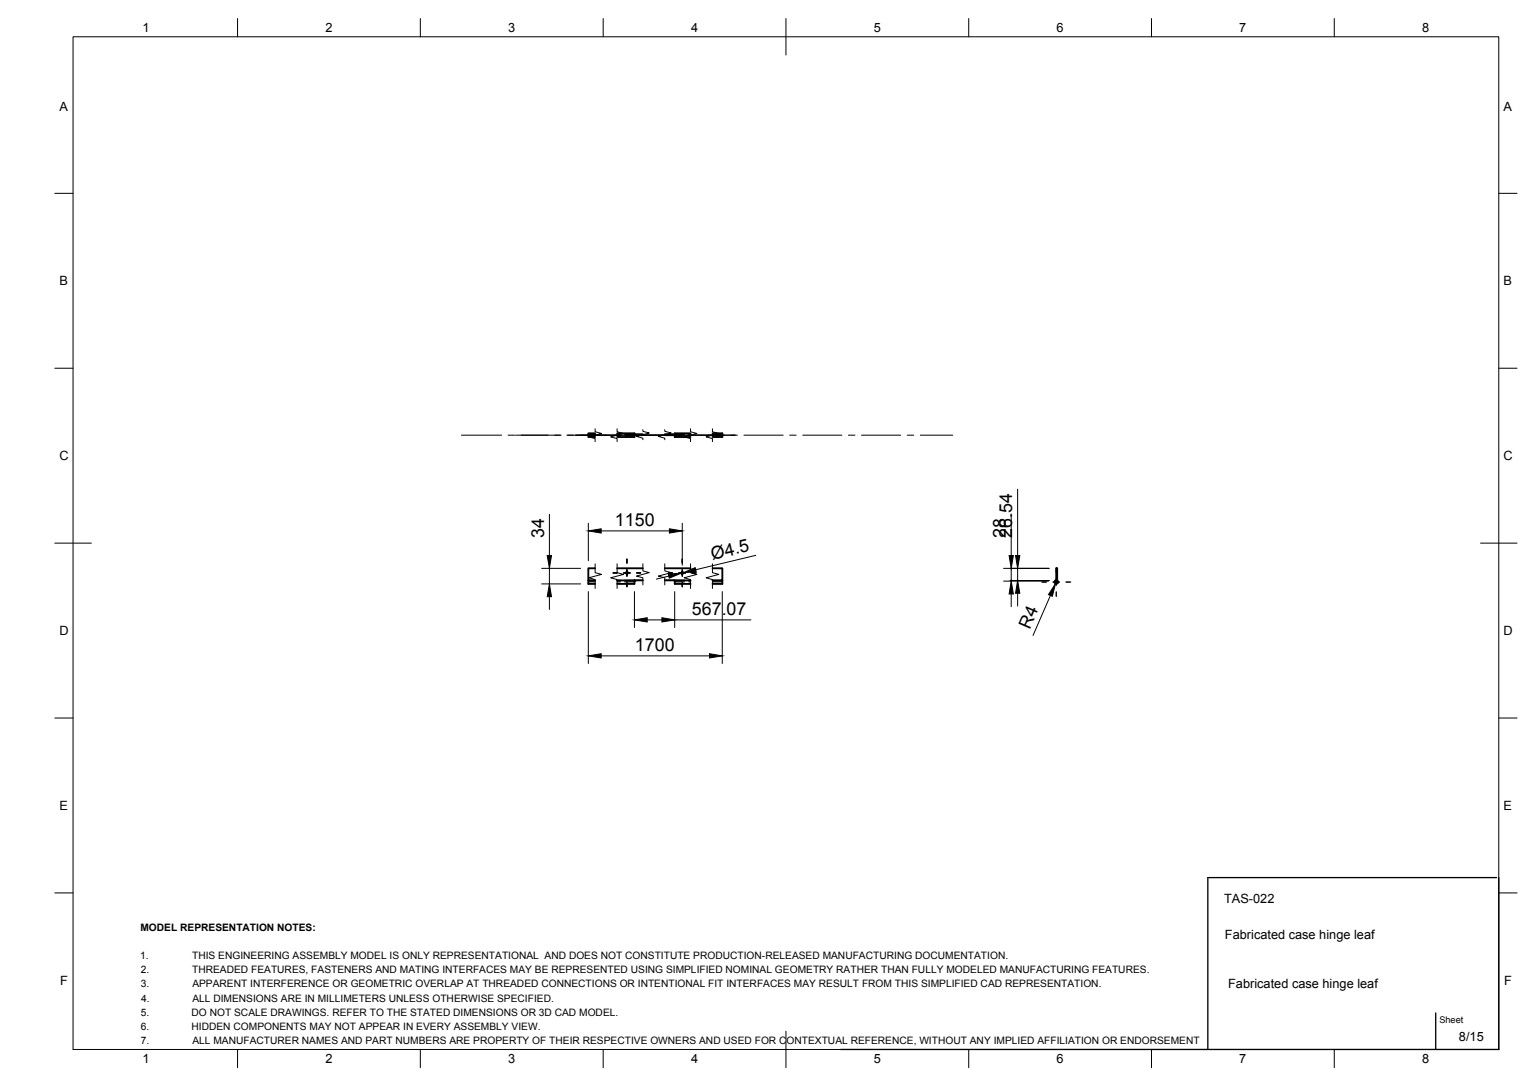
ISO-10303-21;
HEADER;
/* Generated by software containing ST-Developer
 * from STEP Tools, Inc. (www.steptools.com) 
 */

FILE_DESCRIPTION(
/* description */ (''),
/* implementation_level */ '2;1');

FILE_NAME(
/* name */ 'Fabricated case hinge leaf.step',
/* time_stamp */ '2026-11-15T21:02:08-08:00',
/* author */ (''),
/* organization */ (''),
/* preprocessor_version */ 'ST-DEVELOPER v20.2',
/* originating_system */ 'Autodesk Translation Framework v15.17.0.0',
/* authorisation */ '');

FILE_SCHEMA (('AUTOMOTIVE_DESIGN { 1 0 10303 214 3 1 1 }'));
ENDSEC;

DATA;
#10=MECHANICAL_DESIGN_GEOMETRIC_PRESENTATION_REPRESENTATION('',(#604),#31566);
#387=FACE_BOUND('',#931,.T.);
#388=FACE_BOUND('',#932,.T.);
#389=FACE_BOUND('',#939,.T.);
#390=FACE_BOUND('',#941,.T.);
#391=FACE_BOUND('',#942,.T.);
#392=FACE_BOUND('',#948,.T.);
#425=CIRCLE('',#5927,0.225000000000001);
#426=CIRCLE('',#5928,0.225000000000001);
#427=CIRCLE('',#5930,0.224999999999994);
#428=CIRCLE('',#5931,0.224999999999994);
#429=CIRCLE('',#5933,0.42);
#430=CIRCLE('',#5935,0.42);
#431=CIRCLE('',#5941,0.4);
#432=CIRCLE('',#5942,0.22);
#433=CIRCLE('',#5944,0.4);
#434=CIRCLE('',#5946,0.22);
#435=CIRCLE('',#5950,0.22);
#436=CIRCLE('',#5951,0.22);
#437=CIRCLE('',#5953,0.4);
#438=CIRCLE('',#5954,0.4);
#494=CYLINDRICAL_SURFACE('',#5926,0.225000000000001);
#495=CYLINDRICAL_SURFACE('',#5929,0.224999999999994);
#496=CYLINDRICAL_SURFACE('',#5934,0.42);
#497=CYLINDRICAL_SURFACE('',#5943,0.4);
#498=CYLINDRICAL_SURFACE('',#5945,0.22);
#499=CYLINDRICAL_SURFACE('',#5949,0.22);
#500=CYLINDRICAL_SURFACE('',#5952,0.4);
#574=SHAPE_REPRESENTATION_RELATIONSHIP('SRR','None',#31638,#589);
#589=ADVANCED_BREP_SHAPE_REPRESENTATION('',(#619),#31553);
#604=STYLED_ITEM('',(#31720),#619);
#619=MANIFOLD_SOLID_BREP('Body1',#5717);
#650=FACE_OUTER_BOUND('',#925,.T.);
#651=FACE_OUTER_BOUND('',#926,.T.);
#652=FACE_OUTER_BOUND('',#927,.T.);
#653=FACE_OUTER_BOUND('',#928,.T.);
#654=FACE_OUTER_BOUND('',#929,.T.);
#655=FACE_OUTER_BOUND('',#930,.T.);
#656=FACE_OUTER_BOUND('',#933,.T.);
#657=FACE_OUTER_BOUND('',#934,.T.);
#658=FACE_OUTER_BOUND('',#935,.T.);
#659=FACE_OUTER_BOUND('',#936,.T.);
#660=FACE_OUTER_BOUND('',#937,.T.);
#661=FACE_OUTER_BOUND('',#938,.T.);
#662=FACE_OUTER_BOUND('',#940,.T.);
#663=FACE_OUTER_BOUND('',#943,.T.);
#664=FACE_OUTER_BOUND('',#944,.T.);
#665=FACE_OUTER_BOUND('',#945,.T.);
#666=FACE_OUTER_BOUND('',#946,.T.);
#667=FACE_OUTER_BOUND('',#947,.T.);
#925=EDGE_LOOP('',(#3711,#3712,#3713,#3714));
#926=EDGE_LOOP('',(#3715,#3716,#3717,#3718));
#927=EDGE_LOOP('',(#3719,#3720,#3721,#3722));
#928=EDGE_LOOP('',(#3723,#3724,#3725,#3726));
#929=EDGE_LOOP('',(#3727,#3728,#3729,#3730));
#930=EDGE_LOOP('',(#3731,#3732,#3733,#3734,#3735,#3736,#3737,#3738,#3739,
#3740,#3741,#3742));
#931=EDGE_LOOP('',(#3743));
#932=EDGE_LOOP('',(#3744));
#933=EDGE_LOOP('',(#3745,#3746,#3747,#3748,#3749,#3750));
#934=EDGE_LOOP('',(#3751,#3752,#3753,#3754,#3755,#3756));
#935=EDGE_LOOP('',(#3757,#3758,#3759,#3760,#3761));
#936=EDGE_LOOP('',(#3762,#3763,#3764,#3765));
#937=EDGE_LOOP('',(#3766,#3767,#3768,#3769));
#938=EDGE_LOOP('',(#3770,#3771,#3772,#3773));
#939=EDGE_LOOP('',(#3774,#3775,#3776));
#940=EDGE_LOOP('',(#3777,#3778,#3779,#3780,#3781,#3782,#3783,#3784,#3785,
#3786,#3787,#3788,#3789,#3790,#3791,#3792));
#941=EDGE_LOOP('',(#3793));
#942=EDGE_LOOP('',(#3794));
#943=EDGE_LOOP('',(#3795,#3796,#3797,#3798));
#944=EDGE_LOOP('',(#3799,#3800,#3801,#3802));
#945=EDGE_LOOP('',(#3803,#3804,#3805,#3806,#3807));
#946=EDGE_LOOP('',(#3808,#3809,#3810,#3811));
#947=EDGE_LOOP('',(#3812,#3813,#3814,#3815));
#948=EDGE_LOOP('',(#3816,#3817,#3818));
#1240=LINE('',#7657,#1747);
#1241=LINE('',#7663,#1748);
#1242=LINE('',#7668,#1749);
#1243=LINE('',#7672,#1750);
#1244=LINE('',#7673,#1751);
#1245=LINE('',#7676,#1752);
#1246=LINE('',#7679,#1753);
#1247=LINE('',#7682,#1754);
#1248=LINE('',#7684,#1755);
#1249=LINE('',#7685,#1756);
#1250=LINE('',#7688,#1757);
#1251=LINE('',#7690,#1758);
#1252=LINE('',#7692,#1759);
#1253=LINE('',#7694,#1760);
#1254=LINE('',#7696,#1761);
#1255=LINE('',#7698,#1762);
#1256=LINE('',#7700,#1763);
#1257=LINE('',#7702,#1764);
#1258=LINE('',#7703,#1765);
#1259=LINE('',#7706,#1766);
#1260=LINE('',#7708,#1767);
#1261=LINE('',#7710,#1768);
#1262=LINE('',#7711,#1769);
#1263=LINE('',#7714,#1770);
#1264=LINE('',#7716,#1771);
#1265=LINE('',#7718,#1772);
#1266=LINE('',#7719,#1773);
#1267=LINE('',#7724,#1774);
#1268=LINE('',#7729,#1775);
#1269=LINE('',#7732,#1776);
#1270=LINE('',#7736,#1777);
#1271=LINE('',#7737,#1778);
#1272=LINE('',#7738,#1779);
#1273=LINE('',#7741,#1780);
#1274=LINE('',#7743,#1781);
#1275=LINE('',#7745,#1782);
#1276=LINE('',#7747,#1783);
#1277=LINE('',#7749,#1784);
#1278=LINE('',#7750,#1785);
#1279=LINE('',#7759,#1786);
#1747=VECTOR('',#6380,0.225000000000001);
#1748=VECTOR('',#6387,0.224999999999994);
#1749=VECTOR('',#6392,1.);
#1750=VECTOR('',#6395,1.);
#1751=VECTOR('',#6396,1.);
#1752=VECTOR('',#6399,1.);
#1753=VECTOR('',#6402,1.);
#1754=VECTOR('',#6405,1.);
#1755=VECTOR('',#6406,1.);
#1756=VECTOR('',#6407,1.);
#1757=VECTOR('',#6410,1.);
#1758=VECTOR('',#6411,1.);
#1759=VECTOR('',#6412,1.);
#1760=VECTOR('',#6413,1.);
#1761=VECTOR('',#6414,1.);
#1762=VECTOR('',#6415,1.);
#1763=VECTOR('',#6416,1.);
#1764=VECTOR('',#6417,1.);
#1765=VECTOR('',#6418,1.);
#1766=VECTOR('',#6421,1.);
#1767=VECTOR('',#6422,1.);
#1768=VECTOR('',#6423,1.);
#1769=VECTOR('',#6424,1.);
#1770=VECTOR('',#6427,1.);
#1771=VECTOR('',#6428,1.);
#1772=VECTOR('',#6429,1.);
#1773=VECTOR('',#6430,1.);
#1774=VECTOR('',#6435,1.);
#1775=VECTOR('',#6442,1.);
#1776=VECTOR('',#6445,1.);
#1777=VECTOR('',#6450,1.);
#1778=VECTOR('',#6451,1.);
#1779=VECTOR('',#6452,1.);
#1780=VECTOR('',#6455,1.);
#1781=VECTOR('',#6456,1.);
#1782=VECTOR('',#6457,1.);
#1783=VECTOR('',#6458,1.);
#1784=VECTOR('',#6459,1.);
#1785=VECTOR('',#6460,1.);
#1786=VECTOR('',#6477,1.);
#2248=VERTEX_POINT('',#7654);
#2249=VERTEX_POINT('',#7656);
#2250=VERTEX_POINT('',#7660);
#2251=VERTEX_POINT('',#7662);
#2252=VERTEX_POINT('',#7666);
#2253=VERTEX_POINT('',#7667);
#2254=VERTEX_POINT('',#7669);
#2255=VERTEX_POINT('',#7671);
#2256=VERTEX_POINT('',#7675);
#2257=VERTEX_POINT('',#7677);
#2258=VERTEX_POINT('',#7681);
#2259=VERTEX_POINT('',#7683);
#2260=VERTEX_POINT('',#7687);
#2261=VERTEX_POINT('',#7689);
#2262=VERTEX_POINT('',#7691);
#2263=VERTEX_POINT('',#7693);
#2264=VERTEX_POINT('',#7695);
#2265=VERTEX_POINT('',#7697);
#2266=VERTEX_POINT('',#7699);
#2267=VERTEX_POINT('',#7701);
#2268=VERTEX_POINT('',#7705);
#2269=VERTEX_POINT('',#7707);
#2270=VERTEX_POINT('',#7709);
#2271=VERTEX_POINT('',#7713);
#2272=VERTEX_POINT('',#7715);
#2273=VERTEX_POINT('',#7717);
#2274=VERTEX_POINT('',#7721);
#2275=VERTEX_POINT('',#7723);
#2276=VERTEX_POINT('',#7727);
#2277=VERTEX_POINT('',#7731);
#2278=VERTEX_POINT('',#7735);
#2279=VERTEX_POINT('',#7740);
#2280=VERTEX_POINT('',#7742);
#2281=VERTEX_POINT('',#7744);
#2282=VERTEX_POINT('',#7746);
#2283=VERTEX_POINT('',#7748);
#2851=EDGE_CURVE('',#2248,#2248,#425,.T.);
#2852=EDGE_CURVE('',#2248,#2249,#1240,.T.);
#2853=EDGE_CURVE('',#2249,#2249,#426,.T.);
#2854=EDGE_CURVE('',#2250,#2250,#427,.T.);
#2855=EDGE_CURVE('',#2250,#2251,#1241,.T.);
#2856=EDGE_CURVE('',#2251,#2251,#428,.T.);
#2857=EDGE_CURVE('',#2252,#2253,#1242,.T.);
#2858=EDGE_CURVE('',#2254,#2252,#429,.T.);
#2859=EDGE_CURVE('',#2255,#2254,#1243,.T.);
#2860=EDGE_CURVE('',#2253,#2255,#1244,.T.);
#2861=EDGE_CURVE('',#2256,#2252,#1245,.T.);
#2862=EDGE_CURVE('',#2257,#2256,#430,.T.);
#2863=EDGE_CURVE('',#2254,#2257,#1246,.T.);
#2864=EDGE_CURVE('',#2258,#2256,#1247,.T.);
#2865=EDGE_CURVE('',#2259,#2258,#1248,.T.);
#2866=EDGE_CURVE('',#2257,#2259,#1249,.T.);
#2867=EDGE_CURVE('',#2260,#2259,#1250,.T.);
#2868=EDGE_CURVE('',#2260,#2261,#1251,.T.);
#2869=EDGE_CURVE('',#2261,#2262,#1252,.T.);
#2870=EDGE_CURVE('',#2262,#2263,#1253,.T.);
#2871=EDGE_CURVE('',#2263,#2264,#1254,.T.);
#2872=EDGE_CURVE('',#2265,#2264,#1255,.T.);
#2873=EDGE_CURVE('',#2265,#2266,#1256,.T.);
#2874=EDGE_CURVE('',#2266,#2267,#1257,.T.);
#2875=EDGE_CURVE('',#2255,#2267,#1258,.T.);
#2876=EDGE_CURVE('',#2268,#2258,#1259,.T.);
#2877=EDGE_CURVE('',#2268,#2269,#1260,.T.);
#2878=EDGE_CURVE('',#2269,#2270,#1261,.T.);
#2879=EDGE_CURVE('',#2270,#2260,#1262,.T.);
#2880=EDGE_CURVE('',#2267,#2271,#1263,.T.);
#2881=EDGE_CURVE('',#2271,#2272,#1264,.T.);
#2882=EDGE_CURVE('',#2273,#2272,#1265,.T.);
#2883=EDGE_CURVE('',#2253,#2273,#1266,.T.);
#2884=EDGE_CURVE('',#2274,#2266,#431,.T.);
#2885=EDGE_CURVE('',#2275,#2274,#1267,.T.);
#2886=EDGE_CURVE('',#2271,#2275,#432,.T.);
#2887=EDGE_CURVE('',#2276,#2265,#433,.T.);
#2888=EDGE_CURVE('',#2274,#2276,#1268,.T.);
#2889=EDGE_CURVE('',#2277,#2275,#1269,.T.);
#2890=EDGE_CURVE('',#2272,#2277,#434,.T.);
#2891=EDGE_CURVE('',#2264,#2278,#1270,.T.);
#2892=EDGE_CURVE('',#2278,#2276,#1271,.T.);
#2893=EDGE_CURVE('',#2277,#2273,#1272,.T.);
#2894=EDGE_CURVE('',#2279,#2278,#1273,.T.);
#2895=EDGE_CURVE('',#2279,#2280,#1274,.T.);
#2896=EDGE_CURVE('',#2280,#2281,#1275,.T.);
#2897=EDGE_CURVE('',#2281,#2282,#1276,.T.);
#2898=EDGE_CURVE('',#2282,#2283,#1277,.T.);
#2899=EDGE_CURVE('',#2283,#2268,#1278,.T.);
#2900=EDGE_CURVE('',#2269,#2283,#435,.T.);
#2901=EDGE_CURVE('',#2270,#2282,#436,.T.);
#2902=EDGE_CURVE('',#2281,#2261,#437,.T.);
#2903=EDGE_CURVE('',#2280,#2262,#438,.T.);
#2904=EDGE_CURVE('',#2263,#2279,#1279,.T.);
#3711=ORIENTED_EDGE('',*,*,#2851,.F.);
#3712=ORIENTED_EDGE('',*,*,#2852,.T.);
#3713=ORIENTED_EDGE('',*,*,#2853,.F.);
#3714=ORIENTED_EDGE('',*,*,#2852,.F.);
#3715=ORIENTED_EDGE('',*,*,#2854,.F.);
#3716=ORIENTED_EDGE('',*,*,#2855,.T.);
#3717=ORIENTED_EDGE('',*,*,#2856,.F.);
#3718=ORIENTED_EDGE('',*,*,#2855,.F.);
#3719=ORIENTED_EDGE('',*,*,#2857,.F.);
#3720=ORIENTED_EDGE('',*,*,#2858,.F.);
#3721=ORIENTED_EDGE('',*,*,#2859,.F.);
#3722=ORIENTED_EDGE('',*,*,#2860,.F.);
#3723=ORIENTED_EDGE('',*,*,#2861,.F.);
#3724=ORIENTED_EDGE('',*,*,#2862,.F.);
#3725=ORIENTED_EDGE('',*,*,#2863,.F.);
#3726=ORIENTED_EDGE('',*,*,#2858,.T.);
#3727=ORIENTED_EDGE('',*,*,#2864,.F.);
#3728=ORIENTED_EDGE('',*,*,#2865,.F.);
#3729=ORIENTED_EDGE('',*,*,#2866,.F.);
#3730=ORIENTED_EDGE('',*,*,#2862,.T.);
#3731=ORIENTED_EDGE('',*,*,#2859,.T.);
#3732=ORIENTED_EDGE('',*,*,#2863,.T.);
#3733=ORIENTED_EDGE('',*,*,#2866,.T.);
#3734=ORIENTED_EDGE('',*,*,#2867,.F.);
#3735=ORIENTED_EDGE('',*,*,#2868,.T.);
#3736=ORIENTED_EDGE('',*,*,#2869,.T.);
#3737=ORIENTED_EDGE('',*,*,#2870,.T.);
#3738=ORIENTED_EDGE('',*,*,#2871,.T.);
#3739=ORIENTED_EDGE('',*,*,#2872,.F.);
#3740=ORIENTED_EDGE('',*,*,#2873,.T.);
#3741=ORIENTED_EDGE('',*,*,#2874,.T.);
#3742=ORIENTED_EDGE('',*,*,#2875,.F.);
#3743=ORIENTED_EDGE('',*,*,#2853,.T.);
#3744=ORIENTED_EDGE('',*,*,#2856,.T.);
#3745=ORIENTED_EDGE('',*,*,#2865,.T.);
#3746=ORIENTED_EDGE('',*,*,#2876,.F.);
#3747=ORIENTED_EDGE('',*,*,#2877,.T.);
#3748=ORIENTED_EDGE('',*,*,#2878,.T.);
#3749=ORIENTED_EDGE('',*,*,#2879,.T.);
#3750=ORIENTED_EDGE('',*,*,#2867,.T.);
#3751=ORIENTED_EDGE('',*,*,#2860,.T.);
#3752=ORIENTED_EDGE('',*,*,#2875,.T.);
#3753=ORIENTED_EDGE('',*,*,#2880,.T.);
#3754=ORIENTED_EDGE('',*,*,#2881,.T.);
#3755=ORIENTED_EDGE('',*,*,#2882,.F.);
#3756=ORIENTED_EDGE('',*,*,#2883,.F.);
#3757=ORIENTED_EDGE('',*,*,#2880,.F.);
#3758=ORIENTED_EDGE('',*,*,#2874,.F.);
#3759=ORIENTED_EDGE('',*,*,#2884,.F.);
#3760=ORIENTED_EDGE('',*,*,#2885,.F.);
#3761=ORIENTED_EDGE('',*,*,#2886,.F.);
#3762=ORIENTED_EDGE('',*,*,#2873,.F.);
#3763=ORIENTED_EDGE('',*,*,#2887,.F.);
#3764=ORIENTED_EDGE('',*,*,#2888,.F.);
#3765=ORIENTED_EDGE('',*,*,#2884,.T.);
#3766=ORIENTED_EDGE('',*,*,#2881,.F.);
#3767=ORIENTED_EDGE('',*,*,#2886,.T.);
#3768=ORIENTED_EDGE('',*,*,#2889,.F.);
#3769=ORIENTED_EDGE('',*,*,#2890,.F.);
#3770=ORIENTED_EDGE('',*,*,#2872,.T.);
#3771=ORIENTED_EDGE('',*,*,#2891,.T.);
#3772=ORIENTED_EDGE('',*,*,#2892,.T.);
#3773=ORIENTED_EDGE('',*,*,#2887,.T.);
#3774=ORIENTED_EDGE('',*,*,#2890,.T.);
#3775=ORIENTED_EDGE('',*,*,#2893,.T.);
#3776=ORIENTED_EDGE('',*,*,#2882,.T.);
#3777=ORIENTED_EDGE('',*,*,#2857,.T.);
#3778=ORIENTED_EDGE('',*,*,#2883,.T.);
#3779=ORIENTED_EDGE('',*,*,#2893,.F.);
#3780=ORIENTED_EDGE('',*,*,#2889,.T.);
#3781=ORIENTED_EDGE('',*,*,#2885,.T.);
#3782=ORIENTED_EDGE('',*,*,#2888,.T.);
#3783=ORIENTED_EDGE('',*,*,#2892,.F.);
#3784=ORIENTED_EDGE('',*,*,#2894,.F.);
#3785=ORIENTED_EDGE('',*,*,#2895,.T.);
#3786=ORIENTED_EDGE('',*,*,#2896,.T.);
#3787=ORIENTED_EDGE('',*,*,#2897,.T.);
#3788=ORIENTED_EDGE('',*,*,#2898,.T.);
#3789=ORIENTED_EDGE('',*,*,#2899,.T.);
#3790=ORIENTED_EDGE('',*,*,#2876,.T.);
#3791=ORIENTED_EDGE('',*,*,#2864,.T.);
#3792=ORIENTED_EDGE('',*,*,#2861,.T.);
#3793=ORIENTED_EDGE('',*,*,#2851,.T.);
#3794=ORIENTED_EDGE('',*,*,#2854,.T.);
#3795=ORIENTED_EDGE('',*,*,#2878,.F.);
#3796=ORIENTED_EDGE('',*,*,#2900,.T.);
#3797=ORIENTED_EDGE('',*,*,#2898,.F.);
#3798=ORIENTED_EDGE('',*,*,#2901,.F.);
#3799=ORIENTED_EDGE('',*,*,#2869,.F.);
#3800=ORIENTED_EDGE('',*,*,#2902,.F.);
#3801=ORIENTED_EDGE('',*,*,#2896,.F.);
#3802=ORIENTED_EDGE('',*,*,#2903,.T.);
#3803=ORIENTED_EDGE('',*,*,#2879,.F.);
#3804=ORIENTED_EDGE('',*,*,#2901,.T.);
#3805=ORIENTED_EDGE('',*,*,#2897,.F.);
#3806=ORIENTED_EDGE('',*,*,#2902,.T.);
#3807=ORIENTED_EDGE('',*,*,#2868,.F.);
#3808=ORIENTED_EDGE('',*,*,#2904,.T.);
#3809=ORIENTED_EDGE('',*,*,#2894,.T.);
#3810=ORIENTED_EDGE('',*,*,#2891,.F.);
#3811=ORIENTED_EDGE('',*,*,#2871,.F.);
#3812=ORIENTED_EDGE('',*,*,#2903,.F.);
#3813=ORIENTED_EDGE('',*,*,#2895,.F.);
#3814=ORIENTED_EDGE('',*,*,#2904,.F.);
#3815=ORIENTED_EDGE('',*,*,#2870,.F.);
#3816=ORIENTED_EDGE('',*,*,#2877,.F.);
#3817=ORIENTED_EDGE('',*,*,#2899,.F.);
#3818=ORIENTED_EDGE('',*,*,#2900,.F.);
#5277=PLANE('',#5932);
#5278=PLANE('',#5936);
#5279=PLANE('',#5937);
#5280=PLANE('',#5938);
#5281=PLANE('',#5939);
#5282=PLANE('',#5940);
#5283=PLANE('',#5947);
#5284=PLANE('',#5948);
#5285=PLANE('',#5955);
#5286=PLANE('',#5956);
#5287=PLANE('',#5957);
#5464=ADVANCED_FACE('',(#650),#494,.F.);
#5465=ADVANCED_FACE('',(#651),#495,.F.);
#5466=ADVANCED_FACE('',(#652),#5277,.F.);
#5467=ADVANCED_FACE('',(#653),#496,.F.);
#5468=ADVANCED_FACE('',(#654),#5278,.T.);
#5469=ADVANCED_FACE('',(#655,#387,#388),#5279,.T.);
#5470=ADVANCED_FACE('',(#656),#5280,.T.);
#5471=ADVANCED_FACE('',(#657),#5281,.T.);
#5472=ADVANCED_FACE('',(#658),#5282,.F.);
#5473=ADVANCED_FACE('',(#659),#497,.T.);
#5474=ADVANCED_FACE('',(#660),#498,.F.);
#5475=ADVANCED_FACE('',(#661,#389),#5283,.T.);
#5476=ADVANCED_FACE('',(#662,#390,#391),#5284,.T.);
#5477=ADVANCED_FACE('',(#663),#499,.F.);
#5478=ADVANCED_FACE('',(#664),#500,.T.);
#5479=ADVANCED_FACE('',(#665),#5285,.T.);
#5480=ADVANCED_FACE('',(#666),#5286,.T.);
#5481=ADVANCED_FACE('',(#667,#392),#5287,.F.);
#5717=CLOSED_SHELL('',(#5464,#5465,#5466,#5467,#5468,#5469,#5470,#5471,
#5472,#5473,#5474,#5475,#5476,#5477,#5478,#5479,#5480,#5481));
#5925=AXIS2_PLACEMENT_3D('',#7652,#6374,#6375);
#5926=AXIS2_PLACEMENT_3D('',#7653,#6376,#6377);
#5927=AXIS2_PLACEMENT_3D('',#7655,#6378,#6379);
#5928=AXIS2_PLACEMENT_3D('',#7658,#6381,#6382);
#5929=AXIS2_PLACEMENT_3D('',#7659,#6383,#6384);
#5930=AXIS2_PLACEMENT_3D('',#7661,#6385,#6386);
#5931=AXIS2_PLACEMENT_3D('',#7664,#6388,#6389);
#5932=AXIS2_PLACEMENT_3D('',#7665,#6390,#6391);
#5933=AXIS2_PLACEMENT_3D('',#7670,#6393,#6394);
#5934=AXIS2_PLACEMENT_3D('',#7674,#6397,#6398);
#5935=AXIS2_PLACEMENT_3D('',#7678,#6400,#6401);
#5936=AXIS2_PLACEMENT_3D('',#7680,#6403,#6404);
#5937=AXIS2_PLACEMENT_3D('',#7686,#6408,#6409);
#5938=AXIS2_PLACEMENT_3D('',#7704,#6419,#6420);
#5939=AXIS2_PLACEMENT_3D('',#7712,#6425,#6426);
#5940=AXIS2_PLACEMENT_3D('',#7720,#6431,#6432);
#5941=AXIS2_PLACEMENT_3D('',#7722,#6433,#6434);
#5942=AXIS2_PLACEMENT_3D('',#7725,#6436,#6437);
#5943=AXIS2_PLACEMENT_3D('',#7726,#6438,#6439);
#5944=AXIS2_PLACEMENT_3D('',#7728,#6440,#6441);
#5945=AXIS2_PLACEMENT_3D('',#7730,#6443,#6444);
#5946=AXIS2_PLACEMENT_3D('',#7733,#6446,#6447);
#5947=AXIS2_PLACEMENT_3D('',#7734,#6448,#6449);
#5948=AXIS2_PLACEMENT_3D('',#7739,#6453,#6454);
#5949=AXIS2_PLACEMENT_3D('',#7751,#6461,#6462);
#5950=AXIS2_PLACEMENT_3D('',#7752,#6463,#6464);
#5951=AXIS2_PLACEMENT_3D('',#7753,#6465,#6466);
#5952=AXIS2_PLACEMENT_3D('',#7754,#6467,#6468);
#5953=AXIS2_PLACEMENT_3D('',#7755,#6469,#6470);
#5954=AXIS2_PLACEMENT_3D('',#7756,#6471,#6472);
#5955=AXIS2_PLACEMENT_3D('',#7757,#6473,#6474);
#5956=AXIS2_PLACEMENT_3D('',#7758,#6475,#6476);
#5957=AXIS2_PLACEMENT_3D('',#7760,#6478,#6479);
#6374=DIRECTION('axis',(0.,0.,1.));
#6375=DIRECTION('refdir',(1.,0.,0.));
#6376=DIRECTION('center_axis',(1.,0.,0.));
#6377=DIRECTION('ref_axis',(0.,0.,-1.));
#6378=DIRECTION('center_axis',(1.,0.,0.));
#6379=DIRECTION('ref_axis',(0.,0.,-1.));
#6380=DIRECTION('',(1.,0.,0.));
#6381=DIRECTION('center_axis',(-1.,0.,0.));
#6382=DIRECTION('ref_axis',(0.,0.,-1.));
#6383=DIRECTION('center_axis',(1.,0.,0.));
#6384=DIRECTION('ref_axis',(0.,0.,-1.));
#6385=DIRECTION('center_axis',(1.,0.,0.));
#6386=DIRECTION('ref_axis',(0.,0.,-1.));
#6387=DIRECTION('',(1.,0.,0.));
#6388=DIRECTION('center_axis',(-1.,0.,0.));
#6389=DIRECTION('ref_axis',(0.,0.,-1.));
#6390=DIRECTION('center_axis',(0.,0.,1.));
#6391=DIRECTION('ref_axis',(1.,0.,0.));
#6392=DIRECTION('',(0.,-1.,0.));
#6393=DIRECTION('center_axis',(0.,0.,1.));
#6394=DIRECTION('ref_axis',(1.,0.,0.));
#6395=DIRECTION('',(0.,1.,0.));
#6396=DIRECTION('',(1.,0.,0.));
#6397=DIRECTION('center_axis',(0.,0.,1.));
#6398=DIRECTION('ref_axis',(1.,0.,0.));
#6399=DIRECTION('',(0.,0.,1.));
#6400=DIRECTION('center_axis',(0.,0.,1.));
#6401=DIRECTION('ref_axis',(1.,0.,0.));
#6402=DIRECTION('',(0.,0.,-1.));
#6403=DIRECTION('center_axis',(0.,0.,1.));
#6404=DIRECTION('ref_axis',(1.,0.,0.));
#6405=DIRECTION('',(0.,1.,0.));
#6406=DIRECTION('',(-1.,0.,0.));
#6407=DIRECTION('',(0.,-1.,0.));
#6408=DIRECTION('center_axis',(1.,0.,0.));
#6409=DIRECTION('ref_axis',(0.,1.,0.));
#6410=DIRECTION('',(0.,0.,1.));
#6411=DIRECTION('',(0.,1.,0.));
#6412=DIRECTION('',(0.,0.,-1.));
#6413=DIRECTION('',(0.,1.,0.));
#6414=DIRECTION('',(0.,0.,1.));
#6415=DIRECTION('',(0.,1.,0.));
#6416=DIRECTION('',(0.,0.,-1.));
#6417=DIRECTION('',(0.,-1.,0.));
#6418=DIRECTION('',(0.,0.,1.));
#6419=DIRECTION('center_axis',(0.,-1.,0.));
#6420=DIRECTION('ref_axis',(1.,0.,0.));
#6421=DIRECTION('',(0.,0.,1.));
#6422=DIRECTION('',(1.,0.,0.));
#6423=DIRECTION('',(0.,0.,1.));
#6424=DIRECTION('',(1.,0.,0.));
#6425=DIRECTION('center_axis',(0.,-1.,0.));
#6426=DIRECTION('ref_axis',(1.,0.,0.));
#6427=DIRECTION('',(-1.,0.,0.));
#6428=DIRECTION('',(0.,0.,1.));
#6429=DIRECTION('',(1.,0.,0.));
#6430=DIRECTION('',(0.,0.,1.));
#6431=DIRECTION('center_axis',(0.,0.,1.));
#6432=DIRECTION('ref_axis',(1.,0.,0.));
#6433=DIRECTION('center_axis',(0.,0.,1.));
#6434=DIRECTION('ref_axis',(1.,0.,0.));
#6435=DIRECTION('',(0.,1.,0.));
#6436=DIRECTION('center_axis',(0.,0.,-1.));
#6437=DIRECTION('ref_axis',(1.,0.,0.));
#6438=DIRECTION('center_axis',(0.,0.,1.));
#6439=DIRECTION('ref_axis',(-0.25881904510252,-0.965925826289069,0.));
#6440=DIRECTION('center_axis',(0.,0.,1.));
#6441=DIRECTION('ref_axis',(1.,0.,0.));
#6442=DIRECTION('',(0.,0.,1.));
#6443=DIRECTION('center_axis',(0.,0.,1.));
#6444=DIRECTION('ref_axis',(-0.213200716355611,-0.977008420918394,0.));
#6445=DIRECTION('',(0.,0.,-1.));
#6446=DIRECTION('center_axis',(0.,0.,-1.));
#6447=DIRECTION('ref_axis',(1.,0.,0.));
#6448=DIRECTION('center_axis',(0.,0.,1.));
#6449=DIRECTION('ref_axis',(1.,0.,0.));
#6450=DIRECTION('',(-1.,0.,0.));
#6451=DIRECTION('',(0.,-1.,0.));
#6452=DIRECTION('',(0.,-1.,0.));
#6453=DIRECTION('center_axis',(-1.,0.,0.));
#6454=DIRECTION('ref_axis',(0.,-1.,0.));
#6455=DIRECTION('',(0.,0.,1.));
#6456=DIRECTION('',(0.,-1.,0.));
#6457=DIRECTION('',(0.,0.,1.));
#6458=DIRECTION('',(0.,-1.,0.));
#6459=DIRECTION('',(0.,0.,-1.));
#6460=DIRECTION('',(0.,-1.,0.));
#6461=DIRECTION('center_axis',(0.,0.,1.));
#6462=DIRECTION('ref_axis',(-0.213200716355611,-0.977008420918394,0.));
#6463=DIRECTION('center_axis',(0.,0.,-1.));
#6464=DIRECTION('ref_axis',(1.,0.,0.));
#6465=DIRECTION('center_axis',(0.,0.,-1.));
#6466=DIRECTION('ref_axis',(1.,0.,0.));
#6467=DIRECTION('center_axis',(0.,0.,1.));
#6468=DIRECTION('ref_axis',(-0.25881904510252,-0.965925826289069,0.));
#6469=DIRECTION('center_axis',(0.,0.,1.));
#6470=DIRECTION('ref_axis',(1.,0.,0.));
#6471=DIRECTION('center_axis',(0.,0.,1.));
#6472=DIRECTION('ref_axis',(1.,0.,0.));
#6473=DIRECTION('center_axis',(0.,0.,1.));
#6474=DIRECTION('ref_axis',(1.,0.,0.));
#6475=DIRECTION('center_axis',(0.,1.,0.));
#6476=DIRECTION('ref_axis',(-1.,0.,0.));
#6477=DIRECTION('',(-1.,0.,0.));
#6478=DIRECTION('center_axis',(0.,0.,1.));
#6479=DIRECTION('ref_axis',(1.,0.,0.));
#7652=CARTESIAN_POINT('',(0.,0.,0.));
#7653=CARTESIAN_POINT('Origin',(0.,2.,55.));
#7654=CARTESIAN_POINT('',(0.,2.,55.225));
#7655=CARTESIAN_POINT('Origin',(0.,2.,55.));
#7656=CARTESIAN_POINT('',(0.2,2.,55.225));
#7657=CARTESIAN_POINT('',(0.,2.,55.225));
#7658=CARTESIAN_POINT('Origin',(0.2,2.,55.));
#7659=CARTESIAN_POINT('Origin',(0.,2.,115.));
#7660=CARTESIAN_POINT('',(0.,2.,115.225));
#7661=CARTESIAN_POINT('Origin',(0.,2.,115.));
#7662=CARTESIAN_POINT('',(0.2,2.,115.225));
#7663=CARTESIAN_POINT('',(0.,2.,115.225));
#7664=CARTESIAN_POINT('Origin',(0.2,2.,115.));
#7665=CARTESIAN_POINT('Origin',(0.,0.,113.343333333333));
#7666=CARTESIAN_POINT('',(0.,0.42,113.343333333333));
#7667=CARTESIAN_POINT('',(0.,0.2,113.343333333333));
#7668=CARTESIAN_POINT('',(0.,1.5,113.343333333333));
#7669=CARTESIAN_POINT('',(0.2,0.369323706252388,113.343333333333));
#7670=CARTESIAN_POINT('Origin',(0.,0.,113.343333333333));
#7671=CARTESIAN_POINT('',(0.2,0.2,113.343333333333));
#7672=CARTESIAN_POINT('',(0.2,0.1,113.343333333333));
#7673=CARTESIAN_POINT('',(0.,0.2,113.343333333333));
#7674=CARTESIAN_POINT('Origin',(0.,0.,56.6566666666667));
#7675=CARTESIAN_POINT('',(0.,0.42,56.6566666666667));
#7676=CARTESIAN_POINT('',(0.,0.42,56.6566666666667));
#7677=CARTESIAN_POINT('',(0.2,0.369323706252388,56.6566666666667));
#7678=CARTESIAN_POINT('Origin',(0.,0.,56.6566666666667));
#7679=CARTESIAN_POINT('',(0.2,0.369323706252388,56.6566666666667));
#7680=CARTESIAN_POINT('Origin',(0.,0.,56.6566666666667));
#7681=CARTESIAN_POINT('',(0.,0.2,56.6566666666667));
#7682=CARTESIAN_POINT('',(0.,1.5,56.6566666666667));
#7683=CARTESIAN_POINT('',(0.2,0.2,56.6566666666667));
#7684=CARTESIAN_POINT('',(0.,0.2,56.6566666666667));
#7685=CARTESIAN_POINT('',(0.2,0.1,56.6566666666667));
#7686=CARTESIAN_POINT('Origin',(0.2,0.2,0.));
#7687=CARTESIAN_POINT('',(0.2,0.2,56.6466666666667));
#7688=CARTESIAN_POINT('',(0.2,0.2,0.));
#7689=CARTESIAN_POINT('',(0.2,0.346410161513776,56.6466666666667));
#7690=CARTESIAN_POINT('',(0.2,0.1,56.6466666666667));
#7691=CARTESIAN_POINT('',(0.2,0.346410161513776,0.));
#7692=CARTESIAN_POINT('',(0.2,0.346410161513776,0.));
#7693=CARTESIAN_POINT('',(0.2,3.,0.));
#7694=CARTESIAN_POINT('',(0.2,0.2,0.));
#7695=CARTESIAN_POINT('',(0.2,3.,170.));
#7696=CARTESIAN_POINT('',(0.2,3.,0.));
#7697=CARTESIAN_POINT('',(0.2,0.346410161513776,170.));
#7698=CARTESIAN_POINT('',(0.2,0.2,170.));
#7699=CARTESIAN_POINT('',(0.2,0.346410161513776,113.353333333333));
#7700=CARTESIAN_POINT('',(0.2,0.346410161513776,113.353333333333));
#7701=CARTESIAN_POINT('',(0.2,0.2,113.353333333333));
#7702=CARTESIAN_POINT('',(0.2,0.1,113.353333333333));
#7703=CARTESIAN_POINT('',(0.2,0.2,0.));
#7704=CARTESIAN_POINT('Origin',(0.,0.2,0.));
#7705=CARTESIAN_POINT('',(0.,0.2,0.));
#7706=CARTESIAN_POINT('',(0.,0.2,0.));
#7707=CARTESIAN_POINT('',(0.0916515138991168,0.2,0.));
#7708=CARTESIAN_POINT('',(0.,0.2,0.));
#7709=CARTESIAN_POINT('',(0.0916515138991168,0.2,56.6466666666667));
#7710=CARTESIAN_POINT('',(0.0916515138991168,0.2,0.));
#7711=CARTESIAN_POINT('',(0.,0.2,56.6466666666667));
#7712=CARTESIAN_POINT('Origin',(0.,0.2,0.));
#7713=CARTESIAN_POINT('',(0.0916515138991168,0.2,113.353333333333));
#7714=CARTESIAN_POINT('',(0.,0.2,113.353333333333));
#7715=CARTESIAN_POINT('',(0.0916515138991168,0.2,170.));
#7716=CARTESIAN_POINT('',(0.0916515138991168,0.2,113.353333333333));
#7717=CARTESIAN_POINT('',(0.,0.2,170.));
#7718=CARTESIAN_POINT('',(0.,0.2,170.));
#7719=CARTESIAN_POINT('',(0.,0.2,0.));
#7720=CARTESIAN_POINT('Origin',(0.,0.,113.353333333333));
#7721=CARTESIAN_POINT('',(0.,0.4,113.353333333333));
#7722=CARTESIAN_POINT('Origin',(0.,0.,113.353333333333));
#7723=CARTESIAN_POINT('',(0.,0.22,113.353333333333));
#7724=CARTESIAN_POINT('',(0.,1.5,113.353333333333));
#7725=CARTESIAN_POINT('Origin',(0.,0.,113.353333333333));
#7726=CARTESIAN_POINT('Origin',(0.,0.,113.353333333333));
#7727=CARTESIAN_POINT('',(0.,0.4,170.));
#7728=CARTESIAN_POINT('Origin',(0.,0.,170.));
#7729=CARTESIAN_POINT('',(0.,0.4,113.353333333333));
#7730=CARTESIAN_POINT('Origin',(0.,0.,113.353333333333));
#7731=CARTESIAN_POINT('',(0.,0.22,170.));
#7732=CARTESIAN_POINT('',(0.,0.22,113.353333333333));
#7733=CARTESIAN_POINT('Origin',(0.,0.,170.));
#7734=CARTESIAN_POINT('Origin',(0.1,1.6,170.));
#7735=CARTESIAN_POINT('',(0.,3.,170.));
#7736=CARTESIAN_POINT('',(0.2,3.,170.));
#7737=CARTESIAN_POINT('',(0.,3.,170.));
#7738=CARTESIAN_POINT('',(0.,3.,170.));
#7739=CARTESIAN_POINT('Origin',(0.,3.,0.));
#7740=CARTESIAN_POINT('',(0.,3.,0.));
#7741=CARTESIAN_POINT('',(0.,3.,0.));
#7742=CARTESIAN_POINT('',(0.,0.4,0.));
#7743=CARTESIAN_POINT('',(0.,3.,0.));
#7744=CARTESIAN_POINT('',(0.,0.4,56.6466666666667));
#7745=CARTESIAN_POINT('',(0.,0.4,0.));
#7746=CARTESIAN_POINT('',(0.,0.22,56.6466666666667));
#7747=CARTESIAN_POINT('',(0.,1.5,56.6466666666667));
#7748=CARTESIAN_POINT('',(0.,0.22,0.));
#7749=CARTESIAN_POINT('',(0.,0.22,0.));
#7750=CARTESIAN_POINT('',(0.,3.,0.));
#7751=CARTESIAN_POINT('Origin',(0.,0.,0.));
#7752=CARTESIAN_POINT('Origin',(0.,0.,0.));
#7753=CARTESIAN_POINT('Origin',(0.,0.,56.6466666666667));
#7754=CARTESIAN_POINT('Origin',(0.,0.,0.));
#7755=CARTESIAN_POINT('Origin',(0.,0.,56.6466666666667));
#7756=CARTESIAN_POINT('Origin',(0.,0.,0.));
#7757=CARTESIAN_POINT('Origin',(0.,0.,56.6466666666667));
#7758=CARTESIAN_POINT('Origin',(0.2,3.,0.));
#7759=CARTESIAN_POINT('',(0.2,3.,0.));
#7760=CARTESIAN_POINT('Origin',(0.1,1.6,0.));
#31536=UNCERTAINTY_MEASURE_WITH_UNIT(LENGTH_MEASURE(0.001),#31567,
'DISTANCE_ACCURACY_VALUE',
'Maximum model space distance between geometric entities at asserted c
onnectivities');
#31549=UNCERTAINTY_MEASURE_WITH_UNIT(LENGTH_MEASURE(0.001),#31567,
'DISTANCE_ACCURACY_VALUE',
'Maximum model space distance between geometric entities at asserted c
onnectivities');
#31553=(
GEOMETRIC_REPRESENTATION_CONTEXT(3)
GLOBAL_UNCERTAINTY_ASSIGNED_CONTEXT((#31536))
GLOBAL_UNIT_ASSIGNED_CONTEXT((#31567,#31569,#31570))
REPRESENTATION_CONTEXT('','3D')
);
#31566=(
GEOMETRIC_REPRESENTATION_CONTEXT(3)
GLOBAL_UNCERTAINTY_ASSIGNED_CONTEXT((#31549))
GLOBAL_UNIT_ASSIGNED_CONTEXT((#31567,#31569,#31570))
REPRESENTATION_CONTEXT('','3D')
);
#31567=(
LENGTH_UNIT()
NAMED_UNIT(*)
SI_UNIT(.CENTI.,.METRE.)
);
#31569=(
NAMED_UNIT(*)
PLANE_ANGLE_UNIT()
SI_UNIT($,.RADIAN.)
);
#31570=(
NAMED_UNIT(*)
SI_UNIT($,.STERADIAN.)
SOLID_ANGLE_UNIT()
);
#31574=SHAPE_DEFINITION_REPRESENTATION(#31590,#31638);
#31590=PRODUCT_DEFINITION_SHAPE('',$,#31655);
#31638=SHAPE_REPRESENTATION('',(#5925),#31553);
#31651=PRODUCT_DEFINITION_CONTEXT('part definition',#31701,'design');
#31655=PRODUCT_DEFINITION('Fabricated case hinge leaf',
'Fabricated case hinge leaf',#31671,#31651);
#31671=PRODUCT_DEFINITION_FORMATION('',$,#31706);
#31701=APPLICATION_CONTEXT(
'Core Data for Automotive Mechanical Design Process');
#31702=PRODUCT_CONTEXT('part definition',#31701,'mechanical');
#31706=PRODUCT('Fabricated case hinge leaf',
'Fabricated case hinge leaf',$,(#31702));
#31720=PRESENTATION_STYLE_ASSIGNMENT((#31727));
#31727=SURFACE_STYLE_USAGE(.BOTH.,#31734);
#31734=SURFACE_SIDE_STYLE('',(#31741));
#31741=SURFACE_STYLE_FILL_AREA(#31748);
#31748=FILL_AREA_STYLE('Opaque(155,165,179)',(#31755));
#31755=FILL_AREA_STYLE_COLOUR('Opaque(155,165,179)',#31762);
#31762=COLOUR_RGB('Opaque(155,165,179)',0.607843137254902,0.647058823529412,
0.701960784313725);
ENDSEC;
END-ISO-10303-21;
